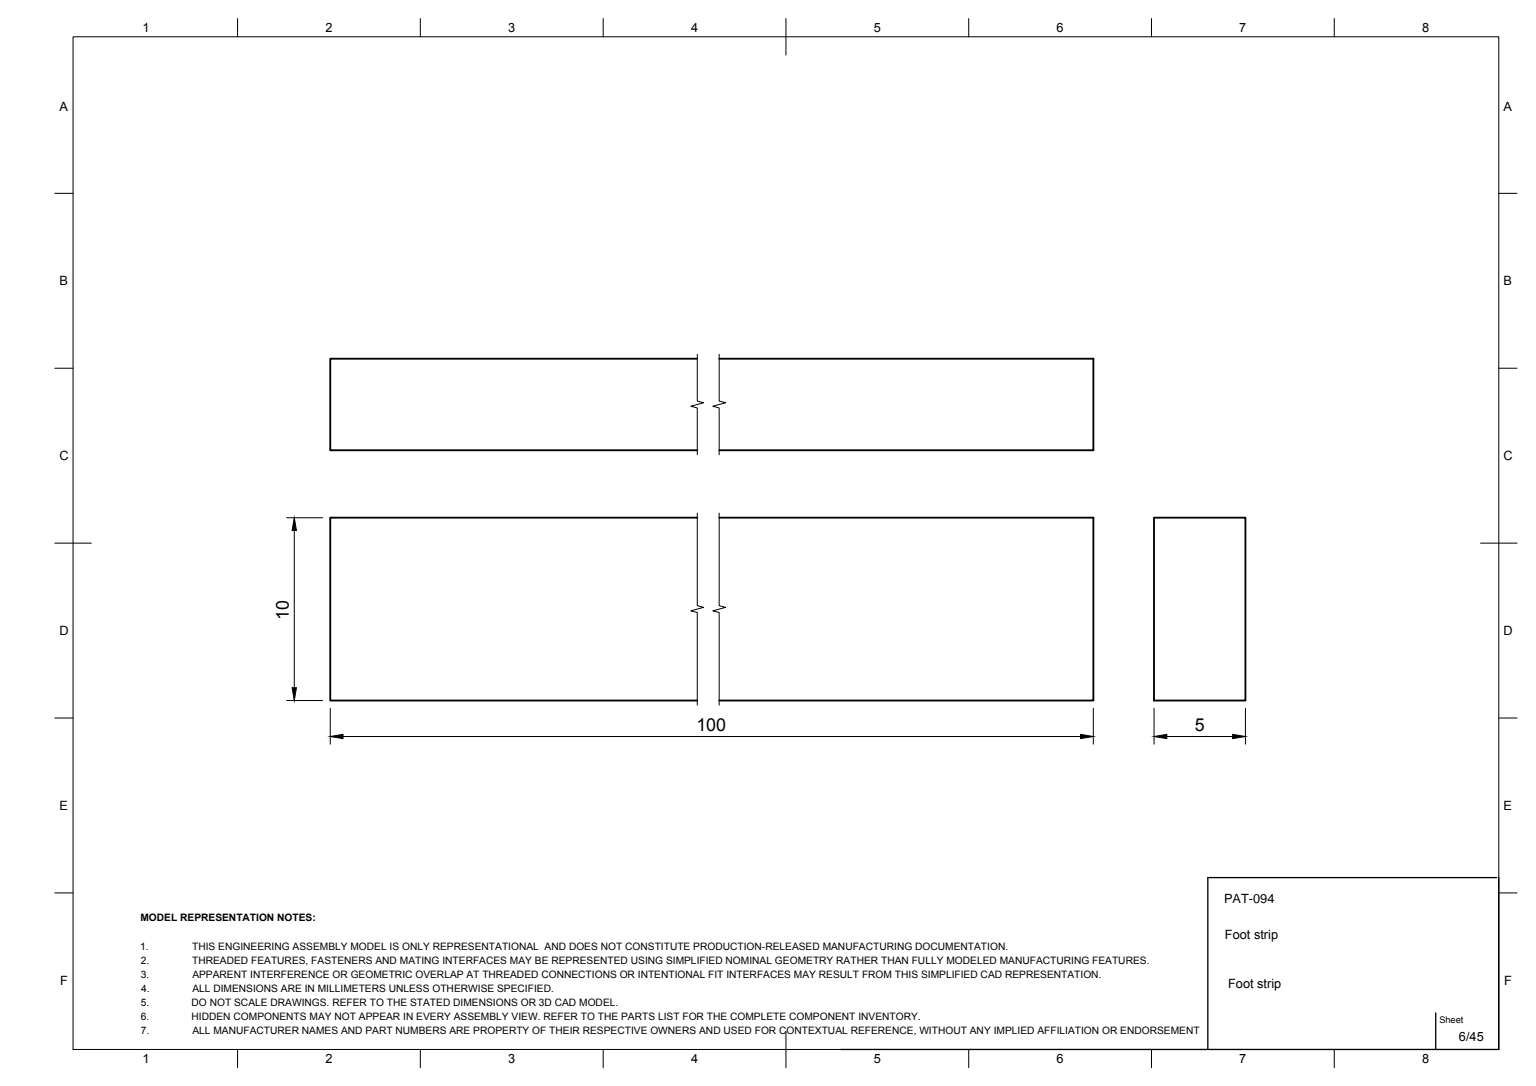
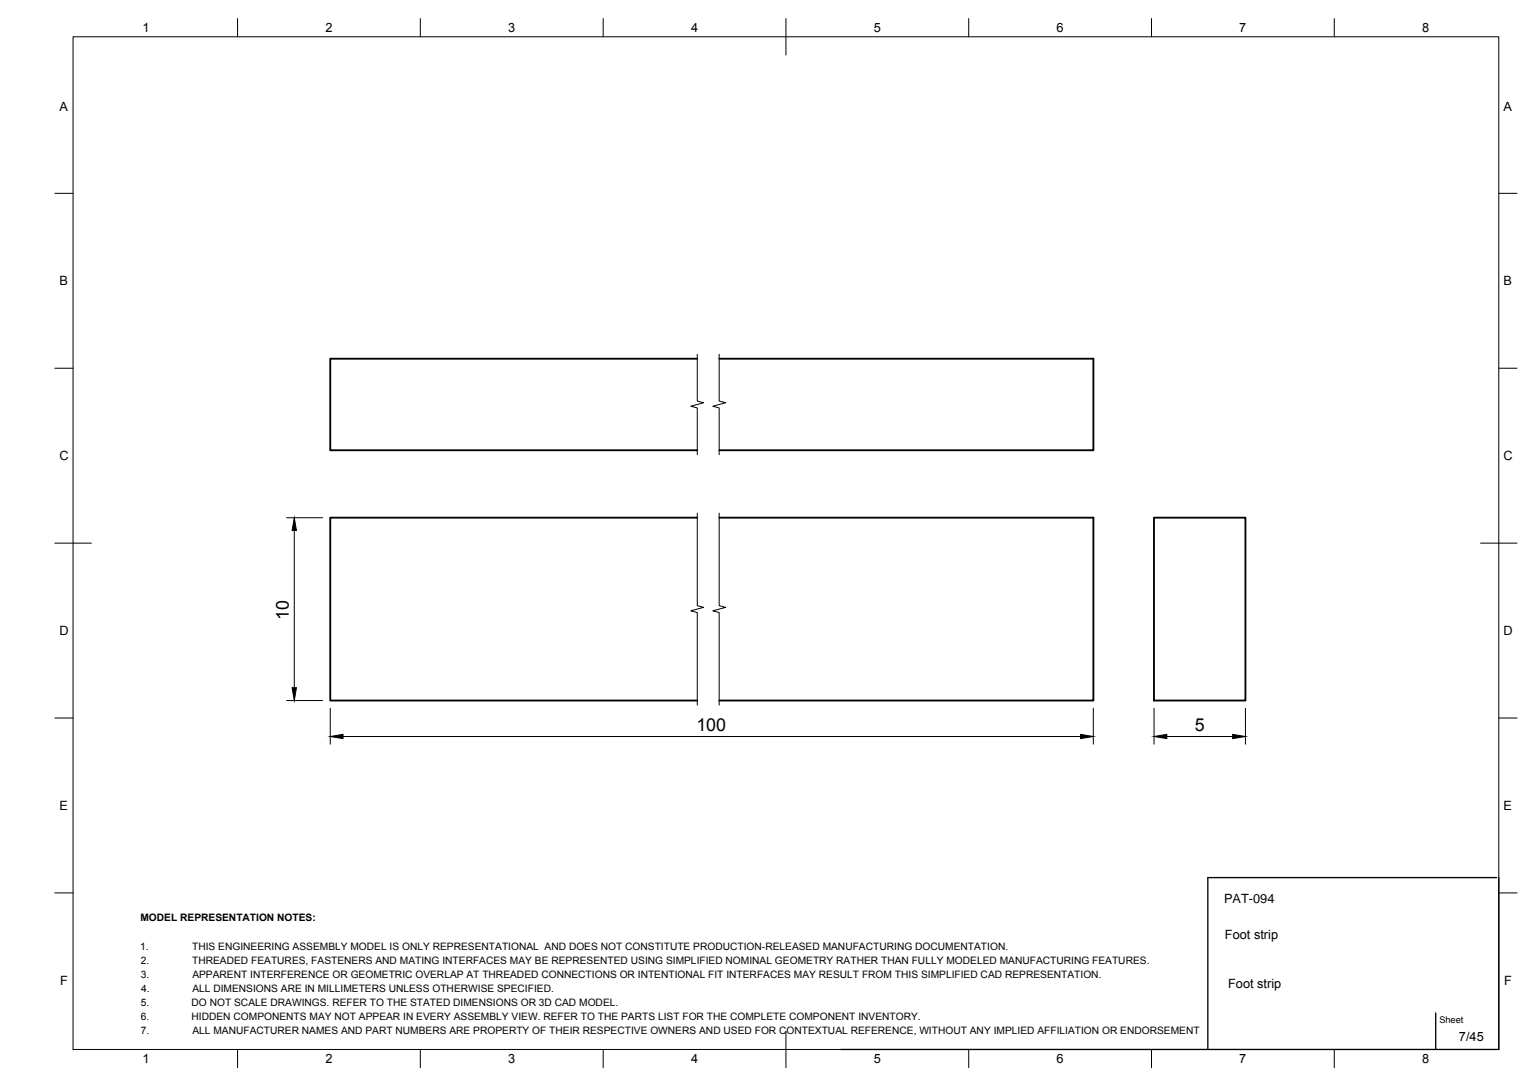
ISO-10303-21;
HEADER;
/* Generated by software containing ST-Developer
 * from STEP Tools, Inc. (www.steptools.com) 
 */

FILE_DESCRIPTION(
/* description */ ('Shaft runout checking stand'),
/* implementation_level */ '2;1');

FILE_NAME(
/* name */ 'Foot strip.step',
/* time_stamp */ '2026-11-02T21:12:33-08:00',
/* author */ (''),
/* organization */ (''),
/* preprocessor_version */ 'ST-DEVELOPER v20.2',
/* originating_system */ 'Autodesk Translation Framework v15.17.0.0',
/* authorisation */ '');

FILE_SCHEMA (('AUTOMOTIVE_DESIGN { 1 0 10303 214 3 1 1 }'));
ENDSEC;

DATA;
#10=MECHANICAL_DESIGN_GEOMETRIC_PRESENTATION_REPRESENTATION('',(#467),#11748);
#381=SHAPE_REPRESENTATION_RELATIONSHIP('SRR','None',#11930,#424);
#424=ADVANCED_BREP_SHAPE_REPRESENTATION('',(#518),#11706);
#467=STYLED_ITEM('',(#12171),#518);
#518=MANIFOLD_SOLID_BREP('Body1',#6210);
#1122=FACE_OUTER_BOUND('',#1519,.T.);
#1123=FACE_OUTER_BOUND('',#1520,.T.);
#1124=FACE_OUTER_BOUND('',#1521,.T.);
#1125=FACE_OUTER_BOUND('',#1522,.T.);
#1126=FACE_OUTER_BOUND('',#1523,.T.);
#1127=FACE_OUTER_BOUND('',#1524,.T.);
#1519=EDGE_LOOP('',(#4548,#4549,#4550,#4551));
#1520=EDGE_LOOP('',(#4552,#4553,#4554,#4555));
#1521=EDGE_LOOP('',(#4556,#4557,#4558,#4559));
#1522=EDGE_LOOP('',(#4560,#4561,#4562,#4563));
#1523=EDGE_LOOP('',(#4564,#4565,#4566,#4567));
#1524=EDGE_LOOP('',(#4568,#4569,#4570,#4571));
#2078=LINE('',#9952,#2545);
#2079=LINE('',#9954,#2546);
#2080=LINE('',#9956,#2547);
#2081=LINE('',#9957,#2548);
#2082=LINE('',#9960,#2549);
#2083=LINE('',#9962,#2550);
#2084=LINE('',#9963,#2551);
#2085=LINE('',#9966,#2552);
#2086=LINE('',#9968,#2553);
#2087=LINE('',#9969,#2554);
#2088=LINE('',#9971,#2555);
#2089=LINE('',#9972,#2556);
#2545=VECTOR('',#7943,1.);
#2546=VECTOR('',#7944,1.);
#2547=VECTOR('',#7945,1.);
#2548=VECTOR('',#7946,1.);
#2549=VECTOR('',#7949,1.);
#2550=VECTOR('',#7950,1.);
#2551=VECTOR('',#7951,1.);
#2552=VECTOR('',#7954,1.);
#2553=VECTOR('',#7955,1.);
#2554=VECTOR('',#7956,1.);
#2555=VECTOR('',#7959,1.);
#2556=VECTOR('',#7960,1.);
#2972=VERTEX_POINT('',#9950);
#2973=VERTEX_POINT('',#9951);
#2974=VERTEX_POINT('',#9953);
#2975=VERTEX_POINT('',#9955);
#2976=VERTEX_POINT('',#9959);
#2977=VERTEX_POINT('',#9961);
#2978=VERTEX_POINT('',#9965);
#2979=VERTEX_POINT('',#9967);
#3560=EDGE_CURVE('',#2972,#2973,#2078,.T.);
#3561=EDGE_CURVE('',#2973,#2974,#2079,.T.);
#3562=EDGE_CURVE('',#2975,#2974,#2080,.T.);
#3563=EDGE_CURVE('',#2972,#2975,#2081,.T.);
#3564=EDGE_CURVE('',#2976,#2972,#2082,.T.);
#3565=EDGE_CURVE('',#2977,#2975,#2083,.T.);
#3566=EDGE_CURVE('',#2976,#2977,#2084,.T.);
#3567=EDGE_CURVE('',#2978,#2976,#2085,.T.);
#3568=EDGE_CURVE('',#2979,#2977,#2086,.T.);
#3569=EDGE_CURVE('',#2978,#2979,#2087,.T.);
#3570=EDGE_CURVE('',#2973,#2978,#2088,.T.);
#3571=EDGE_CURVE('',#2974,#2979,#2089,.T.);
#4548=ORIENTED_EDGE('',*,*,#3560,.T.);
#4549=ORIENTED_EDGE('',*,*,#3561,.T.);
#4550=ORIENTED_EDGE('',*,*,#3562,.F.);
#4551=ORIENTED_EDGE('',*,*,#3563,.F.);
#4552=ORIENTED_EDGE('',*,*,#3564,.T.);
#4553=ORIENTED_EDGE('',*,*,#3563,.T.);
#4554=ORIENTED_EDGE('',*,*,#3565,.F.);
#4555=ORIENTED_EDGE('',*,*,#3566,.F.);
#4556=ORIENTED_EDGE('',*,*,#3567,.T.);
#4557=ORIENTED_EDGE('',*,*,#3566,.T.);
#4558=ORIENTED_EDGE('',*,*,#3568,.F.);
#4559=ORIENTED_EDGE('',*,*,#3569,.F.);
#4560=ORIENTED_EDGE('',*,*,#3570,.T.);
#4561=ORIENTED_EDGE('',*,*,#3569,.T.);
#4562=ORIENTED_EDGE('',*,*,#3571,.F.);
#4563=ORIENTED_EDGE('',*,*,#3561,.F.);
#4564=ORIENTED_EDGE('',*,*,#3571,.T.);
#4565=ORIENTED_EDGE('',*,*,#3568,.T.);
#4566=ORIENTED_EDGE('',*,*,#3565,.T.);
#4567=ORIENTED_EDGE('',*,*,#3562,.T.);
#4568=ORIENTED_EDGE('',*,*,#3570,.F.);
#4569=ORIENTED_EDGE('',*,*,#3560,.F.);
#4570=ORIENTED_EDGE('',*,*,#3564,.F.);
#4571=ORIENTED_EDGE('',*,*,#3567,.F.);
#5671=PLANE('',#6862);
#5672=PLANE('',#6863);
#5673=PLANE('',#6864);
#5674=PLANE('',#6865);
#5675=PLANE('',#6866);
#5676=PLANE('',#6867);
#5922=ADVANCED_FACE('',(#1122),#5671,.T.);
#5923=ADVANCED_FACE('',(#1123),#5672,.T.);
#5924=ADVANCED_FACE('',(#1124),#5673,.T.);
#5925=ADVANCED_FACE('',(#1125),#5674,.T.);
#5926=ADVANCED_FACE('',(#1126),#5675,.T.);
#5927=ADVANCED_FACE('',(#1127),#5676,.F.);
#6210=CLOSED_SHELL('',(#5922,#5923,#5924,#5925,#5926,#5927));
#6861=AXIS2_PLACEMENT_3D('',#9948,#7939,#7940);
#6862=AXIS2_PLACEMENT_3D('',#9949,#7941,#7942);
#6863=AXIS2_PLACEMENT_3D('',#9958,#7947,#7948);
#6864=AXIS2_PLACEMENT_3D('',#9964,#7952,#7953);
#6865=AXIS2_PLACEMENT_3D('',#9970,#7957,#7958);
#6866=AXIS2_PLACEMENT_3D('',#9973,#7961,#7962);
#6867=AXIS2_PLACEMENT_3D('',#9974,#7963,#7964);
#7939=DIRECTION('axis',(0.,0.,1.));
#7940=DIRECTION('refdir',(1.,0.,0.));
#7941=DIRECTION('center_axis',(0.,1.,0.));
#7942=DIRECTION('ref_axis',(-1.,0.,0.));
#7943=DIRECTION('',(-1.,0.,0.));
#7944=DIRECTION('',(0.,0.,1.));
#7945=DIRECTION('',(-1.,0.,0.));
#7946=DIRECTION('',(0.,0.,1.));
#7947=DIRECTION('center_axis',(1.,0.,0.));
#7948=DIRECTION('ref_axis',(0.,1.,0.));
#7949=DIRECTION('',(0.,1.,0.));
#7950=DIRECTION('',(0.,1.,0.));
#7951=DIRECTION('',(0.,0.,1.));
#7952=DIRECTION('center_axis',(0.,-1.,0.));
#7953=DIRECTION('ref_axis',(1.,0.,0.));
#7954=DIRECTION('',(1.,0.,0.));
#7955=DIRECTION('',(1.,0.,0.));
#7956=DIRECTION('',(0.,0.,1.));
#7957=DIRECTION('center_axis',(-1.,0.,0.));
#7958=DIRECTION('ref_axis',(0.,-1.,0.));
#7959=DIRECTION('',(0.,-1.,0.));
#7960=DIRECTION('',(0.,-1.,0.));
#7961=DIRECTION('center_axis',(0.,0.,1.));
#7962=DIRECTION('ref_axis',(1.,0.,0.));
#7963=DIRECTION('center_axis',(0.,0.,1.));
#7964=DIRECTION('ref_axis',(1.,0.,0.));
#9948=CARTESIAN_POINT('',(0.,0.,0.));
#9949=CARTESIAN_POINT('Origin',(5.,-18.,-0.5));
#9950=CARTESIAN_POINT('',(5.,-18.,-0.5));
#9951=CARTESIAN_POINT('',(-5.,-18.,-0.5));
#9952=CARTESIAN_POINT('',(5.,-18.,-0.5));
#9953=CARTESIAN_POINT('',(-5.,-18.,0.));
#9954=CARTESIAN_POINT('',(-5.,-18.,-0.5));
#9955=CARTESIAN_POINT('',(5.,-18.,0.));
#9956=CARTESIAN_POINT('',(5.,-18.,0.));
#9957=CARTESIAN_POINT('',(5.,-18.,-0.5));
#9958=CARTESIAN_POINT('Origin',(5.,-19.,-0.5));
#9959=CARTESIAN_POINT('',(5.,-19.,-0.5));
#9960=CARTESIAN_POINT('',(5.,-19.,-0.5));
#9961=CARTESIAN_POINT('',(5.,-19.,0.));
#9962=CARTESIAN_POINT('',(5.,-19.,0.));
#9963=CARTESIAN_POINT('',(5.,-19.,-0.5));
#9964=CARTESIAN_POINT('Origin',(-5.,-19.,-0.5));
#9965=CARTESIAN_POINT('',(-5.,-19.,-0.5));
#9966=CARTESIAN_POINT('',(-5.,-19.,-0.5));
#9967=CARTESIAN_POINT('',(-5.,-19.,0.));
#9968=CARTESIAN_POINT('',(-5.,-19.,0.));
#9969=CARTESIAN_POINT('',(-5.,-19.,-0.5));
#9970=CARTESIAN_POINT('Origin',(-5.,-18.,-0.5));
#9971=CARTESIAN_POINT('',(-5.,-18.,-0.5));
#9972=CARTESIAN_POINT('',(-5.,-18.,0.));
#9973=CARTESIAN_POINT('Origin',(0.,-18.5,0.));
#9974=CARTESIAN_POINT('Origin',(0.,-18.5,-0.5));
#11657=UNCERTAINTY_MEASURE_WITH_UNIT(LENGTH_MEASURE(0.001),#11749,
'DISTANCE_ACCURACY_VALUE',
'Maximum model space distance between geometric entities at asserted c
onnectivities');
#11699=UNCERTAINTY_MEASURE_WITH_UNIT(LENGTH_MEASURE(0.001),#11749,
'DISTANCE_ACCURACY_VALUE',
'Maximum model space distance between geometric entities at asserted c
onnectivities');
#11706=(
GEOMETRIC_REPRESENTATION_CONTEXT(3)
GLOBAL_UNCERTAINTY_ASSIGNED_CONTEXT((#11657))
GLOBAL_UNIT_ASSIGNED_CONTEXT((#11749,#11751,#11752))
REPRESENTATION_CONTEXT('','3D')
);
#11748=(
GEOMETRIC_REPRESENTATION_CONTEXT(3)
GLOBAL_UNCERTAINTY_ASSIGNED_CONTEXT((#11699))
GLOBAL_UNIT_ASSIGNED_CONTEXT((#11749,#11751,#11752))
REPRESENTATION_CONTEXT('','3D')
);
#11749=(
LENGTH_UNIT()
NAMED_UNIT(*)
SI_UNIT(.CENTI.,.METRE.)
);
#11751=(
NAMED_UNIT(*)
PLANE_ANGLE_UNIT()
SI_UNIT($,.RADIAN.)
);
#11752=(
NAMED_UNIT(*)
SI_UNIT($,.STERADIAN.)
SOLID_ANGLE_UNIT()
);
#11759=SHAPE_DEFINITION_REPRESENTATION(#11807,#11930);
#11807=PRODUCT_DEFINITION_SHAPE('',$,#11979);
#11930=SHAPE_REPRESENTATION('',(#6861),#11706);
#11972=PRODUCT_DEFINITION_CONTEXT('part definition',#12118,'design');
#11979=PRODUCT_DEFINITION('Foot strip','Foot strip',#12027,#11972);
#12027=PRODUCT_DEFINITION_FORMATION('',$,#12126);
#12118=APPLICATION_CONTEXT(
'Core Data for Automotive Mechanical Design Process');
#12119=PRODUCT_CONTEXT('part definition',#12118,'mechanical');
#12126=PRODUCT('Foot strip','Foot strip','Foot strip',(#12119));
#12171=PRESENTATION_STYLE_ASSIGNMENT((#12176));
#12176=SURFACE_STYLE_USAGE(.BOTH.,#12181);
#12181=SURFACE_SIDE_STYLE('',(#12186));
#12186=SURFACE_STYLE_FILL_AREA(#12191);
#12191=FILL_AREA_STYLE('CAD Library Painted - Deep blue',(#12196));
#12196=FILL_AREA_STYLE_COLOUR('CAD Library Painted - Deep blue',#12201);
#12201=COLOUR_RGB('CAD Library Painted - Deep blue',0.0784313725490196,
0.203921568627451,0.349019607843137);
ENDSEC;
END-ISO-10303-21;
